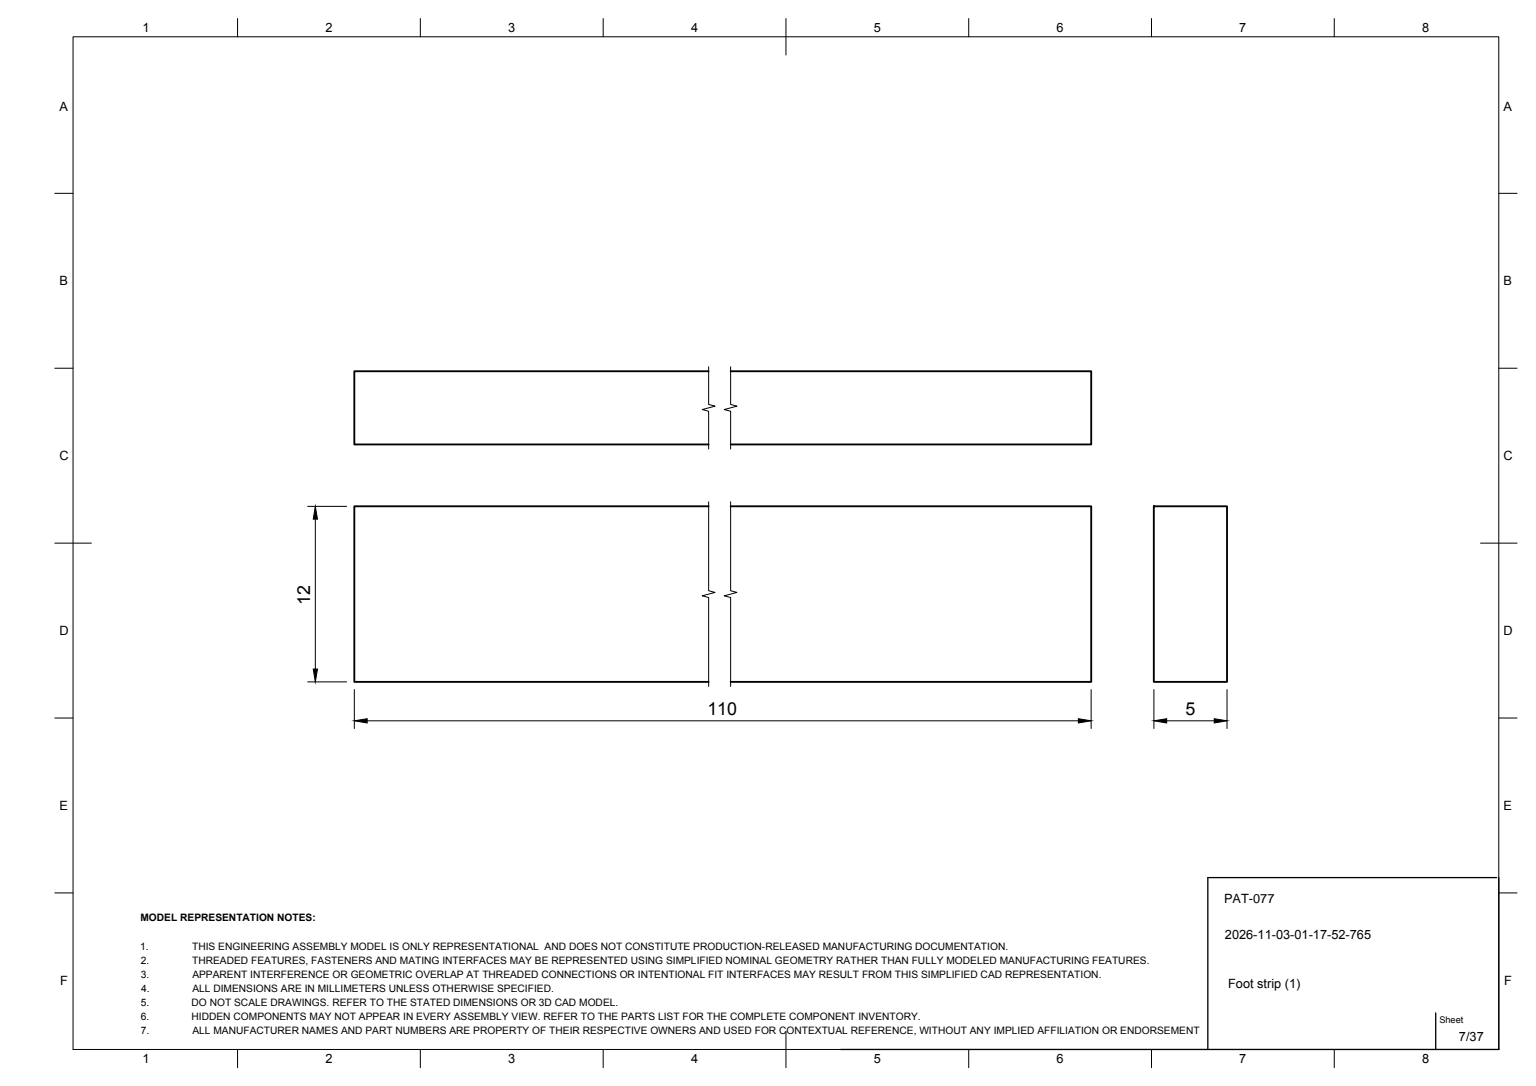
ISO-10303-21;
HEADER;
/* Generated by software containing ST-Developer
 * from STEP Tools, Inc. (www.steptools.com) 
 */

FILE_DESCRIPTION(
/* description */ ('Pallet stop with pneumatic fitting'),
/* implementation_level */ '2;1');

FILE_NAME(
/* name */ 'Foot strip (1).step',
/* time_stamp */ '2026-10-27T10:51:41-07:00',
/* author */ (''),
/* organization */ (''),
/* preprocessor_version */ 'ST-DEVELOPER v20.2',
/* originating_system */ 'Autodesk Translation Framework v15.17.0.0',
/* authorisation */ '');

FILE_SCHEMA (('AUTOMOTIVE_DESIGN { 1 0 10303 214 3 1 1 }'));
ENDSEC;

DATA;
#10=MECHANICAL_DESIGN_GEOMETRIC_PRESENTATION_REPRESENTATION('',(#359),#10265);
#295=SHAPE_REPRESENTATION_RELATIONSHIP('SRR','None',#10408,#327);
#327=ADVANCED_BREP_SHAPE_REPRESENTATION('',(#391),#10232);
#359=STYLED_ITEM('',(#10641),#391);
#391=MANIFOLD_SOLID_BREP('Body1',#5047);
#557=PLANE('',#5476);
#558=PLANE('',#5477);
#559=PLANE('',#5478);
#560=PLANE('',#5479);
#561=PLANE('',#5480);
#562=PLANE('',#5481);
#757=FACE_OUTER_BOUND('',#1089,.T.);
#758=FACE_OUTER_BOUND('',#1090,.T.);
#759=FACE_OUTER_BOUND('',#1091,.T.);
#760=FACE_OUTER_BOUND('',#1092,.T.);
#761=FACE_OUTER_BOUND('',#1093,.T.);
#762=FACE_OUTER_BOUND('',#1094,.T.);
#1089=EDGE_LOOP('',(#3512,#3513,#3514,#3515));
#1090=EDGE_LOOP('',(#3516,#3517,#3518,#3519));
#1091=EDGE_LOOP('',(#3520,#3521,#3522,#3523));
#1092=EDGE_LOOP('',(#3524,#3525,#3526,#3527));
#1093=EDGE_LOOP('',(#3528,#3529,#3530,#3531));
#1094=EDGE_LOOP('',(#3532,#3533,#3534,#3535));
#1523=LINE('',#7852,#1858);
#1524=LINE('',#7854,#1859);
#1525=LINE('',#7856,#1860);
#1526=LINE('',#7857,#1861);
#1527=LINE('',#7860,#1862);
#1528=LINE('',#7862,#1863);
#1529=LINE('',#7863,#1864);
#1530=LINE('',#7866,#1865);
#1531=LINE('',#7868,#1866);
#1532=LINE('',#7869,#1867);
#1533=LINE('',#7871,#1868);
#1534=LINE('',#7872,#1869);
#1858=VECTOR('',#6212,1.);
#1859=VECTOR('',#6213,1.);
#1860=VECTOR('',#6214,1.);
#1861=VECTOR('',#6215,1.);
#1862=VECTOR('',#6218,1.);
#1863=VECTOR('',#6219,1.);
#1864=VECTOR('',#6220,1.);
#1865=VECTOR('',#6223,1.);
#1866=VECTOR('',#6224,1.);
#1867=VECTOR('',#6225,1.);
#1868=VECTOR('',#6228,1.);
#1869=VECTOR('',#6229,1.);
#2441=VERTEX_POINT('',#7850);
#2442=VERTEX_POINT('',#7851);
#2443=VERTEX_POINT('',#7853);
#2444=VERTEX_POINT('',#7855);
#2445=VERTEX_POINT('',#7859);
#2446=VERTEX_POINT('',#7861);
#2447=VERTEX_POINT('',#7865);
#2448=VERTEX_POINT('',#7867);
#2855=EDGE_CURVE('',#2441,#2442,#1523,.T.);
#2856=EDGE_CURVE('',#2442,#2443,#1524,.T.);
#2857=EDGE_CURVE('',#2444,#2443,#1525,.T.);
#2858=EDGE_CURVE('',#2441,#2444,#1526,.T.);
#2859=EDGE_CURVE('',#2445,#2441,#1527,.T.);
#2860=EDGE_CURVE('',#2446,#2444,#1528,.T.);
#2861=EDGE_CURVE('',#2445,#2446,#1529,.T.);
#2862=EDGE_CURVE('',#2447,#2445,#1530,.T.);
#2863=EDGE_CURVE('',#2448,#2446,#1531,.T.);
#2864=EDGE_CURVE('',#2447,#2448,#1532,.T.);
#2865=EDGE_CURVE('',#2442,#2447,#1533,.T.);
#2866=EDGE_CURVE('',#2443,#2448,#1534,.T.);
#3512=ORIENTED_EDGE('',*,*,#2855,.T.);
#3513=ORIENTED_EDGE('',*,*,#2856,.T.);
#3514=ORIENTED_EDGE('',*,*,#2857,.F.);
#3515=ORIENTED_EDGE('',*,*,#2858,.F.);
#3516=ORIENTED_EDGE('',*,*,#2859,.T.);
#3517=ORIENTED_EDGE('',*,*,#2858,.T.);
#3518=ORIENTED_EDGE('',*,*,#2860,.F.);
#3519=ORIENTED_EDGE('',*,*,#2861,.F.);
#3520=ORIENTED_EDGE('',*,*,#2862,.T.);
#3521=ORIENTED_EDGE('',*,*,#2861,.T.);
#3522=ORIENTED_EDGE('',*,*,#2863,.F.);
#3523=ORIENTED_EDGE('',*,*,#2864,.F.);
#3524=ORIENTED_EDGE('',*,*,#2865,.T.);
#3525=ORIENTED_EDGE('',*,*,#2864,.T.);
#3526=ORIENTED_EDGE('',*,*,#2866,.F.);
#3527=ORIENTED_EDGE('',*,*,#2856,.F.);
#3528=ORIENTED_EDGE('',*,*,#2866,.T.);
#3529=ORIENTED_EDGE('',*,*,#2863,.T.);
#3530=ORIENTED_EDGE('',*,*,#2860,.T.);
#3531=ORIENTED_EDGE('',*,*,#2857,.T.);
#3532=ORIENTED_EDGE('',*,*,#2865,.F.);
#3533=ORIENTED_EDGE('',*,*,#2855,.F.);
#3534=ORIENTED_EDGE('',*,*,#2859,.F.);
#3535=ORIENTED_EDGE('',*,*,#2862,.F.);
#4752=ADVANCED_FACE('',(#757),#557,.T.);
#4753=ADVANCED_FACE('',(#758),#558,.T.);
#4754=ADVANCED_FACE('',(#759),#559,.T.);
#4755=ADVANCED_FACE('',(#760),#560,.T.);
#4756=ADVANCED_FACE('',(#761),#561,.T.);
#4757=ADVANCED_FACE('',(#762),#562,.F.);
#5047=CLOSED_SHELL('',(#4752,#4753,#4754,#4755,#4756,#4757));
#5475=AXIS2_PLACEMENT_3D('',#7848,#6208,#6209);
#5476=AXIS2_PLACEMENT_3D('',#7849,#6210,#6211);
#5477=AXIS2_PLACEMENT_3D('',#7858,#6216,#6217);
#5478=AXIS2_PLACEMENT_3D('',#7864,#6221,#6222);
#5479=AXIS2_PLACEMENT_3D('',#7870,#6226,#6227);
#5480=AXIS2_PLACEMENT_3D('',#7873,#6230,#6231);
#5481=AXIS2_PLACEMENT_3D('',#7874,#6232,#6233);
#6208=DIRECTION('axis',(0.,0.,1.));
#6209=DIRECTION('refdir',(1.,0.,0.));
#6210=DIRECTION('center_axis',(0.,1.,0.));
#6211=DIRECTION('ref_axis',(-1.,0.,0.));
#6212=DIRECTION('',(-1.,0.,0.));
#6213=DIRECTION('',(0.,0.,1.));
#6214=DIRECTION('',(-1.,0.,0.));
#6215=DIRECTION('',(0.,0.,1.));
#6216=DIRECTION('center_axis',(1.,0.,0.));
#6217=DIRECTION('ref_axis',(0.,1.,0.));
#6218=DIRECTION('',(0.,1.,0.));
#6219=DIRECTION('',(0.,1.,0.));
#6220=DIRECTION('',(0.,0.,1.));
#6221=DIRECTION('center_axis',(0.,-1.,0.));
#6222=DIRECTION('ref_axis',(1.,0.,0.));
#6223=DIRECTION('',(1.,0.,0.));
#6224=DIRECTION('',(1.,0.,0.));
#6225=DIRECTION('',(0.,0.,1.));
#6226=DIRECTION('center_axis',(-1.,0.,0.));
#6227=DIRECTION('ref_axis',(0.,-1.,0.));
#6228=DIRECTION('',(0.,-1.,0.));
#6229=DIRECTION('',(0.,-1.,0.));
#6230=DIRECTION('center_axis',(0.,0.,1.));
#6231=DIRECTION('ref_axis',(1.,0.,0.));
#6232=DIRECTION('center_axis',(0.,0.,1.));
#6233=DIRECTION('ref_axis',(1.,0.,0.));
#7848=CARTESIAN_POINT('',(0.,0.,0.));
#7849=CARTESIAN_POINT('Origin',(7.5,7.5,-2.2));
#7850=CARTESIAN_POINT('',(7.5,7.5,-2.2));
#7851=CARTESIAN_POINT('',(7.,7.5,-2.2));
#7852=CARTESIAN_POINT('',(7.5,7.5,-2.2));
#7853=CARTESIAN_POINT('',(7.,7.5,-1.));
#7854=CARTESIAN_POINT('',(7.,7.5,-2.2));
#7855=CARTESIAN_POINT('',(7.5,7.5,-1.));
#7856=CARTESIAN_POINT('',(7.5,7.5,-1.));
#7857=CARTESIAN_POINT('',(7.5,7.5,-2.2));
#7858=CARTESIAN_POINT('Origin',(7.5,-3.5,-2.2));
#7859=CARTESIAN_POINT('',(7.5,-3.5,-2.2));
#7860=CARTESIAN_POINT('',(7.5,-3.5,-2.2));
#7861=CARTESIAN_POINT('',(7.5,-3.5,-1.));
#7862=CARTESIAN_POINT('',(7.5,-3.5,-1.));
#7863=CARTESIAN_POINT('',(7.5,-3.5,-2.2));
#7864=CARTESIAN_POINT('Origin',(7.,-3.5,-2.2));
#7865=CARTESIAN_POINT('',(7.,-3.5,-2.2));
#7866=CARTESIAN_POINT('',(7.,-3.5,-2.2));
#7867=CARTESIAN_POINT('',(7.,-3.5,-1.));
#7868=CARTESIAN_POINT('',(7.,-3.5,-1.));
#7869=CARTESIAN_POINT('',(7.,-3.5,-2.2));
#7870=CARTESIAN_POINT('Origin',(7.,7.5,-2.2));
#7871=CARTESIAN_POINT('',(7.,7.5,-2.2));
#7872=CARTESIAN_POINT('',(7.,7.5,-1.));
#7873=CARTESIAN_POINT('Origin',(7.25,2.,-1.));
#7874=CARTESIAN_POINT('Origin',(7.25,2.,-2.2));
#10194=UNCERTAINTY_MEASURE_WITH_UNIT(LENGTH_MEASURE(0.001),#10266,
'DISTANCE_ACCURACY_VALUE',
'Maximum model space distance between geometric entities at asserted c
onnectivities');
#10227=UNCERTAINTY_MEASURE_WITH_UNIT(LENGTH_MEASURE(0.001),#10266,
'DISTANCE_ACCURACY_VALUE',
'Maximum model space distance between geometric entities at asserted c
onnectivities');
#10232=(
GEOMETRIC_REPRESENTATION_CONTEXT(3)
GLOBAL_UNCERTAINTY_ASSIGNED_CONTEXT((#10194))
GLOBAL_UNIT_ASSIGNED_CONTEXT((#10266,#10268,#10269))
REPRESENTATION_CONTEXT('','3D')
);
#10265=(
GEOMETRIC_REPRESENTATION_CONTEXT(3)
GLOBAL_UNCERTAINTY_ASSIGNED_CONTEXT((#10227))
GLOBAL_UNIT_ASSIGNED_CONTEXT((#10266,#10268,#10269))
REPRESENTATION_CONTEXT('','3D')
);
#10266=(
LENGTH_UNIT()
NAMED_UNIT(*)
SI_UNIT(.CENTI.,.METRE.)
);
#10268=(
NAMED_UNIT(*)
PLANE_ANGLE_UNIT()
SI_UNIT($,.RADIAN.)
);
#10269=(
NAMED_UNIT(*)
SI_UNIT($,.STERADIAN.)
SOLID_ANGLE_UNIT()
);
#10274=SHAPE_DEFINITION_REPRESENTATION(#10311,#10408);
#10311=PRODUCT_DEFINITION_SHAPE('',$,#10446);
#10408=SHAPE_REPRESENTATION('',(#5475),#10232);
#10441=PRODUCT_DEFINITION_CONTEXT('part definition',#10554,'design');
#10446=PRODUCT_DEFINITION('Foot strip (1)','Foot strip (1)',#10483,#10441);
#10483=PRODUCT_DEFINITION_FORMATION('',$,#10560);
#10554=APPLICATION_CONTEXT(
'Core Data for Automotive Mechanical Design Process');
#10555=PRODUCT_CONTEXT('part definition',#10554,'mechanical');
#10560=PRODUCT('Foot strip (1)','Foot strip (1)','Foot strip (1)',(#10555));
#10635=COLOUR_RGB('Light Blue',0.38,0.62,0.78);
#10636=FILL_AREA_STYLE_COLOUR('',#10635);
#10637=FILL_AREA_STYLE('',(#10636));
#10638=SURFACE_STYLE_FILL_AREA(#10637);
#10639=SURFACE_SIDE_STYLE('',(#10638));
#10640=SURFACE_STYLE_USAGE(.BOTH.,#10639);
#10641=PRESENTATION_STYLE_ASSIGNMENT((#10640));
ENDSEC;
END-ISO-10303-21;
